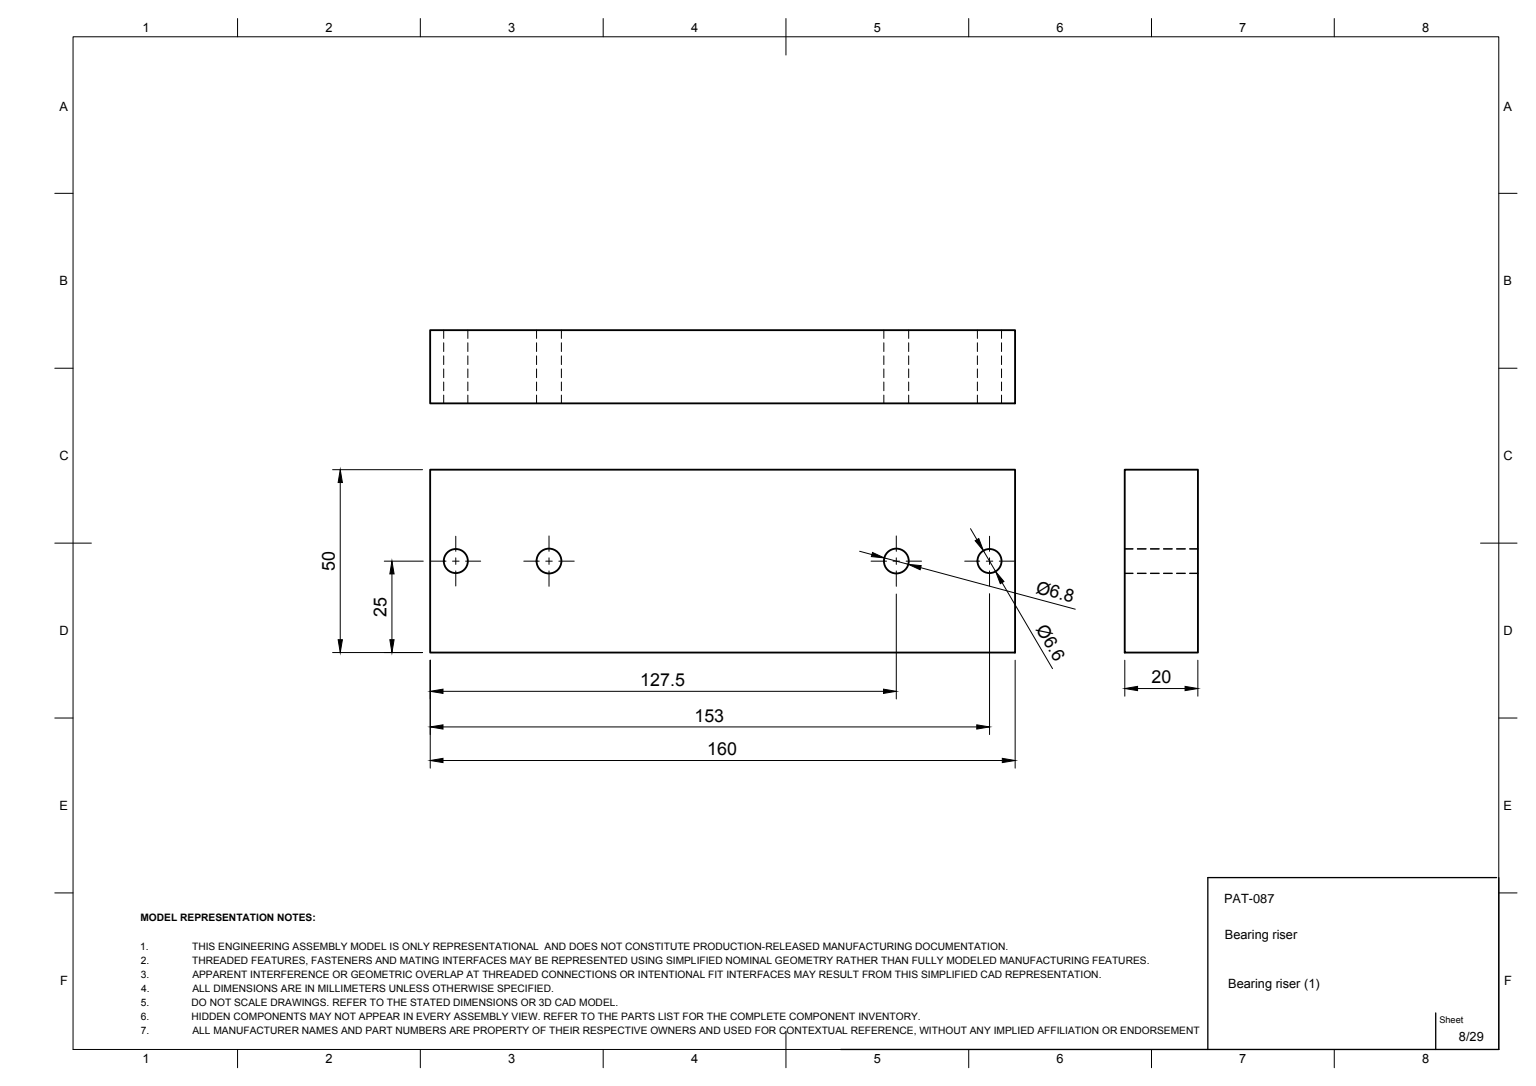
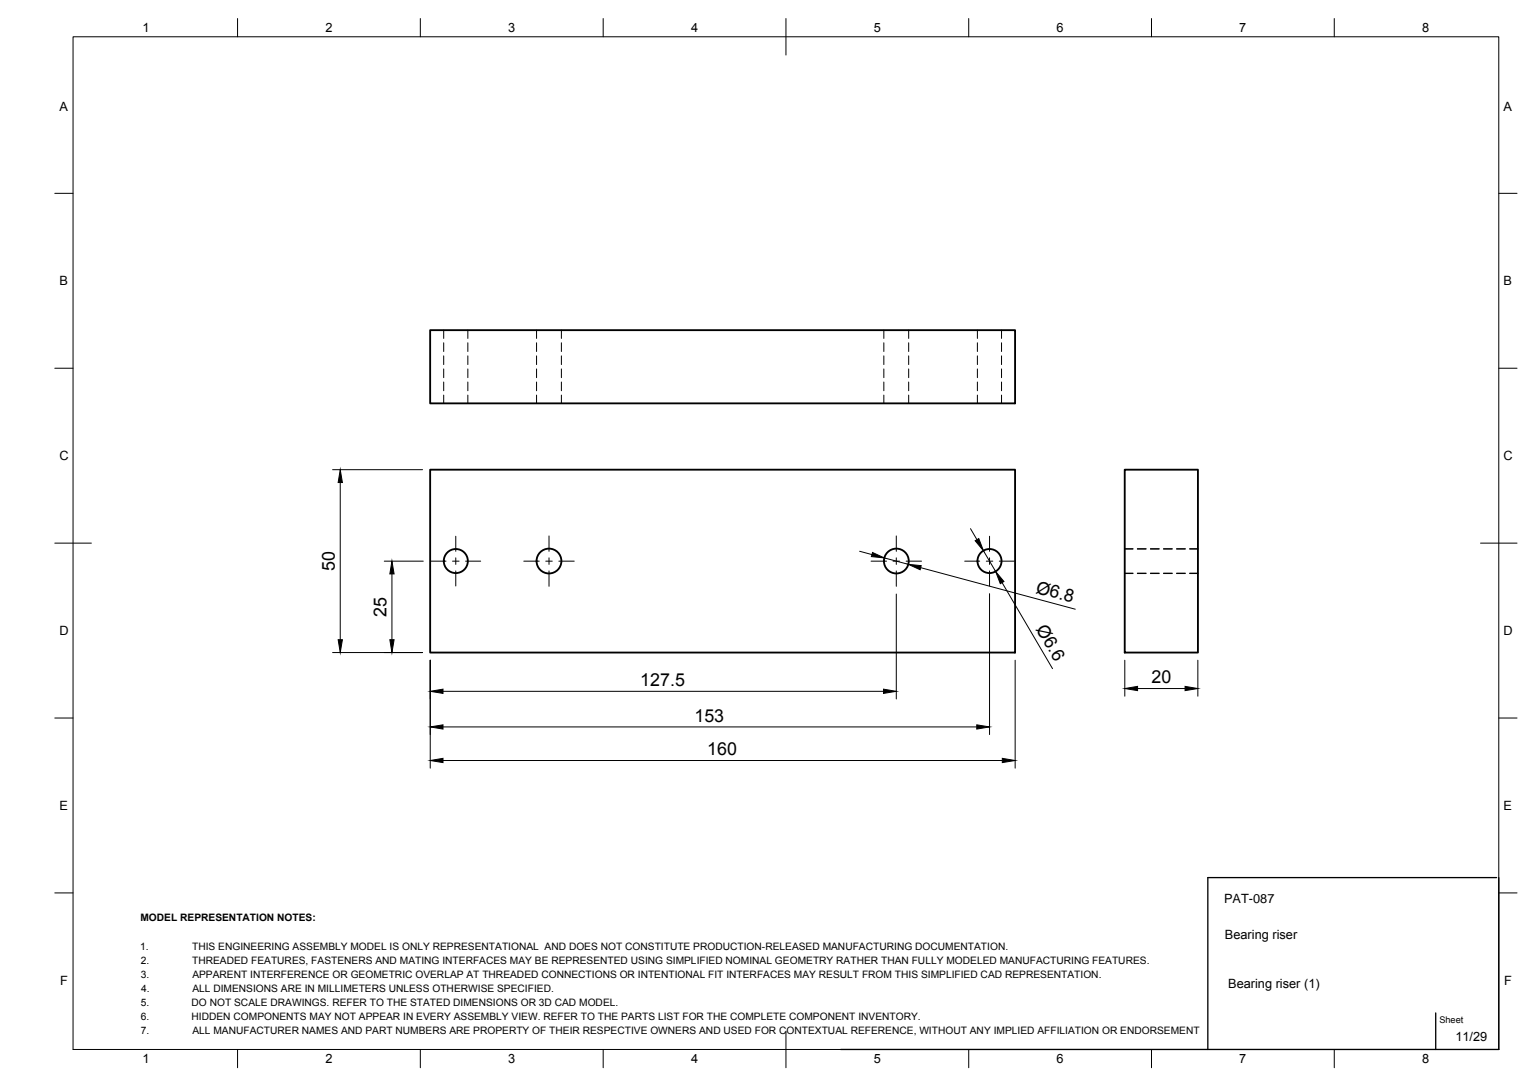
ISO-10303-21;
HEADER;
/* Generated by software containing ST-Developer
 * from STEP Tools, Inc. (www.steptools.com) 
 */

FILE_DESCRIPTION(
/* description */ ('Rigid flange shaft coupling assembly'),
/* implementation_level */ '2;1');

FILE_NAME(
/* name */ 'Bearing riser (1).step',
/* time_stamp */ '2026-10-27T10:47:16-07:00',
/* author */ (''),
/* organization */ (''),
/* preprocessor_version */ 'ST-DEVELOPER v20.2',
/* originating_system */ 'Autodesk Translation Framework v15.17.0.0',
/* authorisation */ '');

FILE_SCHEMA (('AUTOMOTIVE_DESIGN { 1 0 10303 214 3 1 1 }'));
ENDSEC;

DATA;
#10=MECHANICAL_DESIGN_GEOMETRIC_PRESENTATION_REPRESENTATION('',(#404),#9141);
#348=SHAPE_REPRESENTATION_RELATIONSHIP('SRR','None',#9282,#376);
#376=ADVANCED_BREP_SHAPE_REPRESENTATION('',(#433),#9117);
#404=STYLED_ITEM('',(#9500),#433);
#433=MANIFOLD_SOLID_BREP('Body1',#4758);
#473=FACE_BOUND('',#1085,.T.);
#474=FACE_BOUND('',#1086,.T.);
#475=FACE_BOUND('',#1087,.T.);
#476=FACE_BOUND('',#1088,.T.);
#477=FACE_BOUND('',#1090,.T.);
#478=FACE_BOUND('',#1091,.T.);
#479=FACE_BOUND('',#1092,.T.);
#480=FACE_BOUND('',#1093,.T.);
#598=PLANE('',#5178);
#599=PLANE('',#5179);
#600=PLANE('',#5180);
#601=PLANE('',#5181);
#602=PLANE('',#5182);
#603=PLANE('',#5183);
#784=FACE_OUTER_BOUND('',#1076,.T.);
#785=FACE_OUTER_BOUND('',#1077,.T.);
#786=FACE_OUTER_BOUND('',#1078,.T.);
#787=FACE_OUTER_BOUND('',#1079,.T.);
#788=FACE_OUTER_BOUND('',#1080,.T.);
#789=FACE_OUTER_BOUND('',#1081,.T.);
#790=FACE_OUTER_BOUND('',#1082,.T.);
#791=FACE_OUTER_BOUND('',#1083,.T.);
#792=FACE_OUTER_BOUND('',#1084,.T.);
#793=FACE_OUTER_BOUND('',#1089,.T.);
#1076=EDGE_LOOP('',(#3411,#3412,#3413,#3414));
#1077=EDGE_LOOP('',(#3415,#3416,#3417,#3418));
#1078=EDGE_LOOP('',(#3419,#3420,#3421,#3422));
#1079=EDGE_LOOP('',(#3423,#3424,#3425,#3426));
#1080=EDGE_LOOP('',(#3427,#3428,#3429,#3430));
#1081=EDGE_LOOP('',(#3431,#3432,#3433,#3434));
#1082=EDGE_LOOP('',(#3435,#3436,#3437,#3438));
#1083=EDGE_LOOP('',(#3439,#3440,#3441,#3442));
#1084=EDGE_LOOP('',(#3443,#3444,#3445,#3446));
#1085=EDGE_LOOP('',(#3447));
#1086=EDGE_LOOP('',(#3448));
#1087=EDGE_LOOP('',(#3449));
#1088=EDGE_LOOP('',(#3450));
#1089=EDGE_LOOP('',(#3451,#3452,#3453,#3454));
#1090=EDGE_LOOP('',(#3455));
#1091=EDGE_LOOP('',(#3456));
#1092=EDGE_LOOP('',(#3457));
#1093=EDGE_LOOP('',(#3458));
#1465=LINE('',#7278,#1810);
#1466=LINE('',#7284,#1811);
#1467=LINE('',#7290,#1812);
#1468=LINE('',#7296,#1813);
#1469=LINE('',#7301,#1814);
#1470=LINE('',#7303,#1815);
#1471=LINE('',#7305,#1816);
#1472=LINE('',#7306,#1817);
#1473=LINE('',#7309,#1818);
#1474=LINE('',#7311,#1819);
#1475=LINE('',#7312,#1820);
#1476=LINE('',#7315,#1821);
#1477=LINE('',#7317,#1822);
#1478=LINE('',#7318,#1823);
#1479=LINE('',#7320,#1824);
#1480=LINE('',#7321,#1825);
#1810=VECTOR('',#5852,0.34);
#1811=VECTOR('',#5859,0.34);
#1812=VECTOR('',#5866,0.33);
#1813=VECTOR('',#5873,0.33);
#1814=VECTOR('',#5878,1.);
#1815=VECTOR('',#5879,1.);
#1816=VECTOR('',#5880,1.);
#1817=VECTOR('',#5881,1.);
#1818=VECTOR('',#5884,1.);
#1819=VECTOR('',#5885,1.);
#1820=VECTOR('',#5886,1.);
#1821=VECTOR('',#5889,1.);
#1822=VECTOR('',#5890,1.);
#1823=VECTOR('',#5891,1.);
#1824=VECTOR('',#5894,1.);
#1825=VECTOR('',#5895,1.);
#2119=CIRCLE('',#5167,0.34);
#2120=CIRCLE('',#5168,0.34);
#2121=CIRCLE('',#5170,0.34);
#2122=CIRCLE('',#5171,0.34);
#2123=CIRCLE('',#5173,0.33);
#2124=CIRCLE('',#5174,0.33);
#2125=CIRCLE('',#5176,0.33);
#2126=CIRCLE('',#5177,0.33);
#2332=VERTEX_POINT('',#7275);
#2333=VERTEX_POINT('',#7277);
#2334=VERTEX_POINT('',#7281);
#2335=VERTEX_POINT('',#7283);
#2336=VERTEX_POINT('',#7287);
#2337=VERTEX_POINT('',#7289);
#2338=VERTEX_POINT('',#7293);
#2339=VERTEX_POINT('',#7295);
#2340=VERTEX_POINT('',#7299);
#2341=VERTEX_POINT('',#7300);
#2342=VERTEX_POINT('',#7302);
#2343=VERTEX_POINT('',#7304);
#2344=VERTEX_POINT('',#7308);
#2345=VERTEX_POINT('',#7310);
#2346=VERTEX_POINT('',#7314);
#2347=VERTEX_POINT('',#7316);
#2749=EDGE_CURVE('',#2332,#2332,#2119,.T.);
#2750=EDGE_CURVE('',#2332,#2333,#1465,.T.);
#2751=EDGE_CURVE('',#2333,#2333,#2120,.T.);
#2752=EDGE_CURVE('',#2334,#2334,#2121,.T.);
#2753=EDGE_CURVE('',#2334,#2335,#1466,.T.);
#2754=EDGE_CURVE('',#2335,#2335,#2122,.T.);
#2755=EDGE_CURVE('',#2336,#2336,#2123,.T.);
#2756=EDGE_CURVE('',#2336,#2337,#1467,.T.);
#2757=EDGE_CURVE('',#2337,#2337,#2124,.T.);
#2758=EDGE_CURVE('',#2338,#2338,#2125,.T.);
#2759=EDGE_CURVE('',#2338,#2339,#1468,.T.);
#2760=EDGE_CURVE('',#2339,#2339,#2126,.T.);
#2761=EDGE_CURVE('',#2340,#2341,#1469,.T.);
#2762=EDGE_CURVE('',#2341,#2342,#1470,.T.);
#2763=EDGE_CURVE('',#2343,#2342,#1471,.T.);
#2764=EDGE_CURVE('',#2340,#2343,#1472,.T.);
#2765=EDGE_CURVE('',#2344,#2340,#1473,.T.);
#2766=EDGE_CURVE('',#2345,#2343,#1474,.T.);
#2767=EDGE_CURVE('',#2344,#2345,#1475,.T.);
#2768=EDGE_CURVE('',#2346,#2344,#1476,.T.);
#2769=EDGE_CURVE('',#2347,#2345,#1477,.T.);
#2770=EDGE_CURVE('',#2346,#2347,#1478,.T.);
#2771=EDGE_CURVE('',#2341,#2346,#1479,.T.);
#2772=EDGE_CURVE('',#2342,#2347,#1480,.T.);
#3411=ORIENTED_EDGE('',*,*,#2749,.F.);
#3412=ORIENTED_EDGE('',*,*,#2750,.T.);
#3413=ORIENTED_EDGE('',*,*,#2751,.F.);
#3414=ORIENTED_EDGE('',*,*,#2750,.F.);
#3415=ORIENTED_EDGE('',*,*,#2752,.F.);
#3416=ORIENTED_EDGE('',*,*,#2753,.T.);
#3417=ORIENTED_EDGE('',*,*,#2754,.F.);
#3418=ORIENTED_EDGE('',*,*,#2753,.F.);
#3419=ORIENTED_EDGE('',*,*,#2755,.F.);
#3420=ORIENTED_EDGE('',*,*,#2756,.T.);
#3421=ORIENTED_EDGE('',*,*,#2757,.F.);
#3422=ORIENTED_EDGE('',*,*,#2756,.F.);
#3423=ORIENTED_EDGE('',*,*,#2758,.F.);
#3424=ORIENTED_EDGE('',*,*,#2759,.T.);
#3425=ORIENTED_EDGE('',*,*,#2760,.F.);
#3426=ORIENTED_EDGE('',*,*,#2759,.F.);
#3427=ORIENTED_EDGE('',*,*,#2761,.T.);
#3428=ORIENTED_EDGE('',*,*,#2762,.T.);
#3429=ORIENTED_EDGE('',*,*,#2763,.F.);
#3430=ORIENTED_EDGE('',*,*,#2764,.F.);
#3431=ORIENTED_EDGE('',*,*,#2765,.T.);
#3432=ORIENTED_EDGE('',*,*,#2764,.T.);
#3433=ORIENTED_EDGE('',*,*,#2766,.F.);
#3434=ORIENTED_EDGE('',*,*,#2767,.F.);
#3435=ORIENTED_EDGE('',*,*,#2768,.T.);
#3436=ORIENTED_EDGE('',*,*,#2767,.T.);
#3437=ORIENTED_EDGE('',*,*,#2769,.F.);
#3438=ORIENTED_EDGE('',*,*,#2770,.F.);
#3439=ORIENTED_EDGE('',*,*,#2771,.T.);
#3440=ORIENTED_EDGE('',*,*,#2770,.T.);
#3441=ORIENTED_EDGE('',*,*,#2772,.F.);
#3442=ORIENTED_EDGE('',*,*,#2762,.F.);
#3443=ORIENTED_EDGE('',*,*,#2772,.T.);
#3444=ORIENTED_EDGE('',*,*,#2769,.T.);
#3445=ORIENTED_EDGE('',*,*,#2766,.T.);
#3446=ORIENTED_EDGE('',*,*,#2763,.T.);
#3447=ORIENTED_EDGE('',*,*,#2751,.T.);
#3448=ORIENTED_EDGE('',*,*,#2754,.T.);
#3449=ORIENTED_EDGE('',*,*,#2757,.T.);
#3450=ORIENTED_EDGE('',*,*,#2760,.T.);
#3451=ORIENTED_EDGE('',*,*,#2771,.F.);
#3452=ORIENTED_EDGE('',*,*,#2761,.F.);
#3453=ORIENTED_EDGE('',*,*,#2765,.F.);
#3454=ORIENTED_EDGE('',*,*,#2768,.F.);
#3455=ORIENTED_EDGE('',*,*,#2749,.T.);
#3456=ORIENTED_EDGE('',*,*,#2752,.T.);
#3457=ORIENTED_EDGE('',*,*,#2755,.T.);
#3458=ORIENTED_EDGE('',*,*,#2758,.T.);
#4411=CYLINDRICAL_SURFACE('',#5166,0.34);
#4412=CYLINDRICAL_SURFACE('',#5169,0.34);
#4413=CYLINDRICAL_SURFACE('',#5172,0.33);
#4414=CYLINDRICAL_SURFACE('',#5175,0.33);
#4520=ADVANCED_FACE('',(#784),#4411,.F.);
#4521=ADVANCED_FACE('',(#785),#4412,.F.);
#4522=ADVANCED_FACE('',(#786),#4413,.F.);
#4523=ADVANCED_FACE('',(#787),#4414,.F.);
#4524=ADVANCED_FACE('',(#788),#598,.T.);
#4525=ADVANCED_FACE('',(#789),#599,.T.);
#4526=ADVANCED_FACE('',(#790),#600,.T.);
#4527=ADVANCED_FACE('',(#791),#601,.T.);
#4528=ADVANCED_FACE('',(#792,#473,#474,#475,#476),#602,.T.);
#4529=ADVANCED_FACE('',(#793,#477,#478,#479,#480),#603,.F.);
#4758=CLOSED_SHELL('',(#4520,#4521,#4522,#4523,#4524,#4525,#4526,#4527,
#4528,#4529));
#5165=AXIS2_PLACEMENT_3D('',#7273,#5846,#5847);
#5166=AXIS2_PLACEMENT_3D('',#7274,#5848,#5849);
#5167=AXIS2_PLACEMENT_3D('',#7276,#5850,#5851);
#5168=AXIS2_PLACEMENT_3D('',#7279,#5853,#5854);
#5169=AXIS2_PLACEMENT_3D('',#7280,#5855,#5856);
#5170=AXIS2_PLACEMENT_3D('',#7282,#5857,#5858);
#5171=AXIS2_PLACEMENT_3D('',#7285,#5860,#5861);
#5172=AXIS2_PLACEMENT_3D('',#7286,#5862,#5863);
#5173=AXIS2_PLACEMENT_3D('',#7288,#5864,#5865);
#5174=AXIS2_PLACEMENT_3D('',#7291,#5867,#5868);
#5175=AXIS2_PLACEMENT_3D('',#7292,#5869,#5870);
#5176=AXIS2_PLACEMENT_3D('',#7294,#5871,#5872);
#5177=AXIS2_PLACEMENT_3D('',#7297,#5874,#5875);
#5178=AXIS2_PLACEMENT_3D('',#7298,#5876,#5877);
#5179=AXIS2_PLACEMENT_3D('',#7307,#5882,#5883);
#5180=AXIS2_PLACEMENT_3D('',#7313,#5887,#5888);
#5181=AXIS2_PLACEMENT_3D('',#7319,#5892,#5893);
#5182=AXIS2_PLACEMENT_3D('',#7322,#5896,#5897);
#5183=AXIS2_PLACEMENT_3D('',#7323,#5898,#5899);
#5846=DIRECTION('axis',(0.,0.,1.));
#5847=DIRECTION('refdir',(1.,0.,0.));
#5848=DIRECTION('center_axis',(0.,0.,1.));
#5849=DIRECTION('ref_axis',(1.,0.,0.));
#5850=DIRECTION('center_axis',(0.,0.,1.));
#5851=DIRECTION('ref_axis',(1.,0.,0.));
#5852=DIRECTION('',(0.,0.,1.));
#5853=DIRECTION('center_axis',(0.,0.,-1.));
#5854=DIRECTION('ref_axis',(1.,0.,0.));
#5855=DIRECTION('center_axis',(0.,0.,1.));
#5856=DIRECTION('ref_axis',(1.,0.,0.));
#5857=DIRECTION('center_axis',(0.,0.,1.));
#5858=DIRECTION('ref_axis',(1.,0.,0.));
#5859=DIRECTION('',(0.,0.,1.));
#5860=DIRECTION('center_axis',(0.,0.,-1.));
#5861=DIRECTION('ref_axis',(1.,0.,0.));
#5862=DIRECTION('center_axis',(0.,0.,1.));
#5863=DIRECTION('ref_axis',(1.,0.,0.));
#5864=DIRECTION('center_axis',(0.,0.,1.));
#5865=DIRECTION('ref_axis',(1.,0.,0.));
#5866=DIRECTION('',(0.,0.,1.));
#5867=DIRECTION('center_axis',(0.,0.,-1.));
#5868=DIRECTION('ref_axis',(1.,0.,0.));
#5869=DIRECTION('center_axis',(0.,0.,1.));
#5870=DIRECTION('ref_axis',(1.,0.,0.));
#5871=DIRECTION('center_axis',(0.,0.,1.));
#5872=DIRECTION('ref_axis',(1.,0.,0.));
#5873=DIRECTION('',(0.,0.,1.));
#5874=DIRECTION('center_axis',(0.,0.,-1.));
#5875=DIRECTION('ref_axis',(1.,0.,0.));
#5876=DIRECTION('center_axis',(0.,1.,0.));
#5877=DIRECTION('ref_axis',(-1.,0.,0.));
#5878=DIRECTION('',(-1.,0.,0.));
#5879=DIRECTION('',(0.,0.,1.));
#5880=DIRECTION('',(-1.,0.,0.));
#5881=DIRECTION('',(0.,0.,1.));
#5882=DIRECTION('center_axis',(1.,0.,0.));
#5883=DIRECTION('ref_axis',(0.,1.,0.));
#5884=DIRECTION('',(0.,1.,0.));
#5885=DIRECTION('',(0.,1.,0.));
#5886=DIRECTION('',(0.,0.,1.));
#5887=DIRECTION('center_axis',(0.,-1.,0.));
#5888=DIRECTION('ref_axis',(1.,0.,0.));
#5889=DIRECTION('',(1.,0.,0.));
#5890=DIRECTION('',(1.,0.,0.));
#5891=DIRECTION('',(0.,0.,1.));
#5892=DIRECTION('center_axis',(-1.,0.,0.));
#5893=DIRECTION('ref_axis',(0.,-1.,0.));
#5894=DIRECTION('',(0.,-1.,0.));
#5895=DIRECTION('',(0.,-1.,0.));
#5896=DIRECTION('center_axis',(0.,0.,1.));
#5897=DIRECTION('ref_axis',(1.,0.,0.));
#5898=DIRECTION('center_axis',(0.,0.,1.));
#5899=DIRECTION('ref_axis',(1.,0.,0.));
#7273=CARTESIAN_POINT('',(0.,0.,0.));
#7274=CARTESIAN_POINT('Origin',(-4.75,20.,1.1));
#7275=CARTESIAN_POINT('',(-5.09,20.,1.2));
#7276=CARTESIAN_POINT('Origin',(-4.75,20.,1.2));
#7277=CARTESIAN_POINT('',(-5.09,20.,3.2));
#7278=CARTESIAN_POINT('',(-5.09,20.,1.1));
#7279=CARTESIAN_POINT('Origin',(-4.75,20.,3.2));
#7280=CARTESIAN_POINT('Origin',(4.75,20.,1.1));
#7281=CARTESIAN_POINT('',(4.41,20.,1.2));
#7282=CARTESIAN_POINT('Origin',(4.75,20.,1.2));
#7283=CARTESIAN_POINT('',(4.41,20.,3.2));
#7284=CARTESIAN_POINT('',(4.41,20.,1.1));
#7285=CARTESIAN_POINT('Origin',(4.75,20.,3.2));
#7286=CARTESIAN_POINT('Origin',(-7.3,20.,1.1));
#7287=CARTESIAN_POINT('',(-7.63,20.,1.2));
#7288=CARTESIAN_POINT('Origin',(-7.3,20.,1.2));
#7289=CARTESIAN_POINT('',(-7.63,20.,3.2));
#7290=CARTESIAN_POINT('',(-7.63,20.,1.1));
#7291=CARTESIAN_POINT('Origin',(-7.3,20.,3.2));
#7292=CARTESIAN_POINT('Origin',(7.3,20.,1.1));
#7293=CARTESIAN_POINT('',(6.97,20.,1.2));
#7294=CARTESIAN_POINT('Origin',(7.3,20.,1.2));
#7295=CARTESIAN_POINT('',(6.97,20.,3.2));
#7296=CARTESIAN_POINT('',(6.97,20.,1.1));
#7297=CARTESIAN_POINT('Origin',(7.3,20.,3.2));
#7298=CARTESIAN_POINT('Origin',(8.,22.5,1.2));
#7299=CARTESIAN_POINT('',(8.,22.5,1.2));
#7300=CARTESIAN_POINT('',(-8.,22.5,1.2));
#7301=CARTESIAN_POINT('',(8.,22.5,1.2));
#7302=CARTESIAN_POINT('',(-8.,22.5,3.2));
#7303=CARTESIAN_POINT('',(-8.,22.5,1.2));
#7304=CARTESIAN_POINT('',(8.,22.5,3.2));
#7305=CARTESIAN_POINT('',(8.,22.5,3.2));
#7306=CARTESIAN_POINT('',(8.,22.5,1.2));
#7307=CARTESIAN_POINT('Origin',(8.,17.5,1.2));
#7308=CARTESIAN_POINT('',(8.,17.5,1.2));
#7309=CARTESIAN_POINT('',(8.,17.5,1.2));
#7310=CARTESIAN_POINT('',(8.,17.5,3.2));
#7311=CARTESIAN_POINT('',(8.,17.5,3.2));
#7312=CARTESIAN_POINT('',(8.,17.5,1.2));
#7313=CARTESIAN_POINT('Origin',(-8.,17.5,1.2));
#7314=CARTESIAN_POINT('',(-8.,17.5,1.2));
#7315=CARTESIAN_POINT('',(-8.,17.5,1.2));
#7316=CARTESIAN_POINT('',(-8.,17.5,3.2));
#7317=CARTESIAN_POINT('',(-8.,17.5,3.2));
#7318=CARTESIAN_POINT('',(-8.,17.5,1.2));
#7319=CARTESIAN_POINT('Origin',(-8.,22.5,1.2));
#7320=CARTESIAN_POINT('',(-8.,22.5,1.2));
#7321=CARTESIAN_POINT('',(-8.,22.5,3.2));
#7322=CARTESIAN_POINT('Origin',(0.,20.,3.2));
#7323=CARTESIAN_POINT('Origin',(0.,20.,1.2));
#9084=UNCERTAINTY_MEASURE_WITH_UNIT(LENGTH_MEASURE(0.001),#9142,
'DISTANCE_ACCURACY_VALUE',
'Maximum model space distance between geometric entities at asserted c
onnectivities');
#9108=UNCERTAINTY_MEASURE_WITH_UNIT(LENGTH_MEASURE(0.001),#9142,
'DISTANCE_ACCURACY_VALUE',
'Maximum model space distance between geometric entities at asserted c
onnectivities');
#9117=(
GEOMETRIC_REPRESENTATION_CONTEXT(3)
GLOBAL_UNCERTAINTY_ASSIGNED_CONTEXT((#9084))
GLOBAL_UNIT_ASSIGNED_CONTEXT((#9142,#9144,#9145))
REPRESENTATION_CONTEXT('','3D')
);
#9141=(
GEOMETRIC_REPRESENTATION_CONTEXT(3)
GLOBAL_UNCERTAINTY_ASSIGNED_CONTEXT((#9108))
GLOBAL_UNIT_ASSIGNED_CONTEXT((#9142,#9144,#9145))
REPRESENTATION_CONTEXT('','3D')
);
#9142=(
LENGTH_UNIT()
NAMED_UNIT(*)
SI_UNIT(.CENTI.,.METRE.)
);
#9144=(
NAMED_UNIT(*)
PLANE_ANGLE_UNIT()
SI_UNIT($,.RADIAN.)
);
#9145=(
NAMED_UNIT(*)
SI_UNIT($,.STERADIAN.)
SOLID_ANGLE_UNIT()
);
#9154=SHAPE_DEFINITION_REPRESENTATION(#9186,#9282);
#9186=PRODUCT_DEFINITION_SHAPE('',$,#9315);
#9282=SHAPE_REPRESENTATION('',(#5165),#9117);
#9306=PRODUCT_DEFINITION_CONTEXT('part definition',#9404,'design');
#9315=PRODUCT_DEFINITION('Bearing riser (1)','Bearing riser (1)',#9347,#9306);
#9347=PRODUCT_DEFINITION_FORMATION('',$,#9414);
#9404=APPLICATION_CONTEXT(
'Core Data for Automotive Mechanical Design Process');
#9405=PRODUCT_CONTEXT('part definition',#9404,'mechanical');
#9414=PRODUCT('Bearing riser (1)','Bearing riser (1)','Bearing riser (1)',(#9405));
#9494=COLOUR_RGB('Grey',0.48,0.52,0.57);
#9495=FILL_AREA_STYLE_COLOUR('',#9494);
#9496=FILL_AREA_STYLE('',(#9495));
#9497=SURFACE_STYLE_FILL_AREA(#9496);
#9498=SURFACE_SIDE_STYLE('',(#9497));
#9499=SURFACE_STYLE_USAGE(.BOTH.,#9498);
#9500=PRESENTATION_STYLE_ASSIGNMENT((#9499));
ENDSEC;
END-ISO-10303-21;
